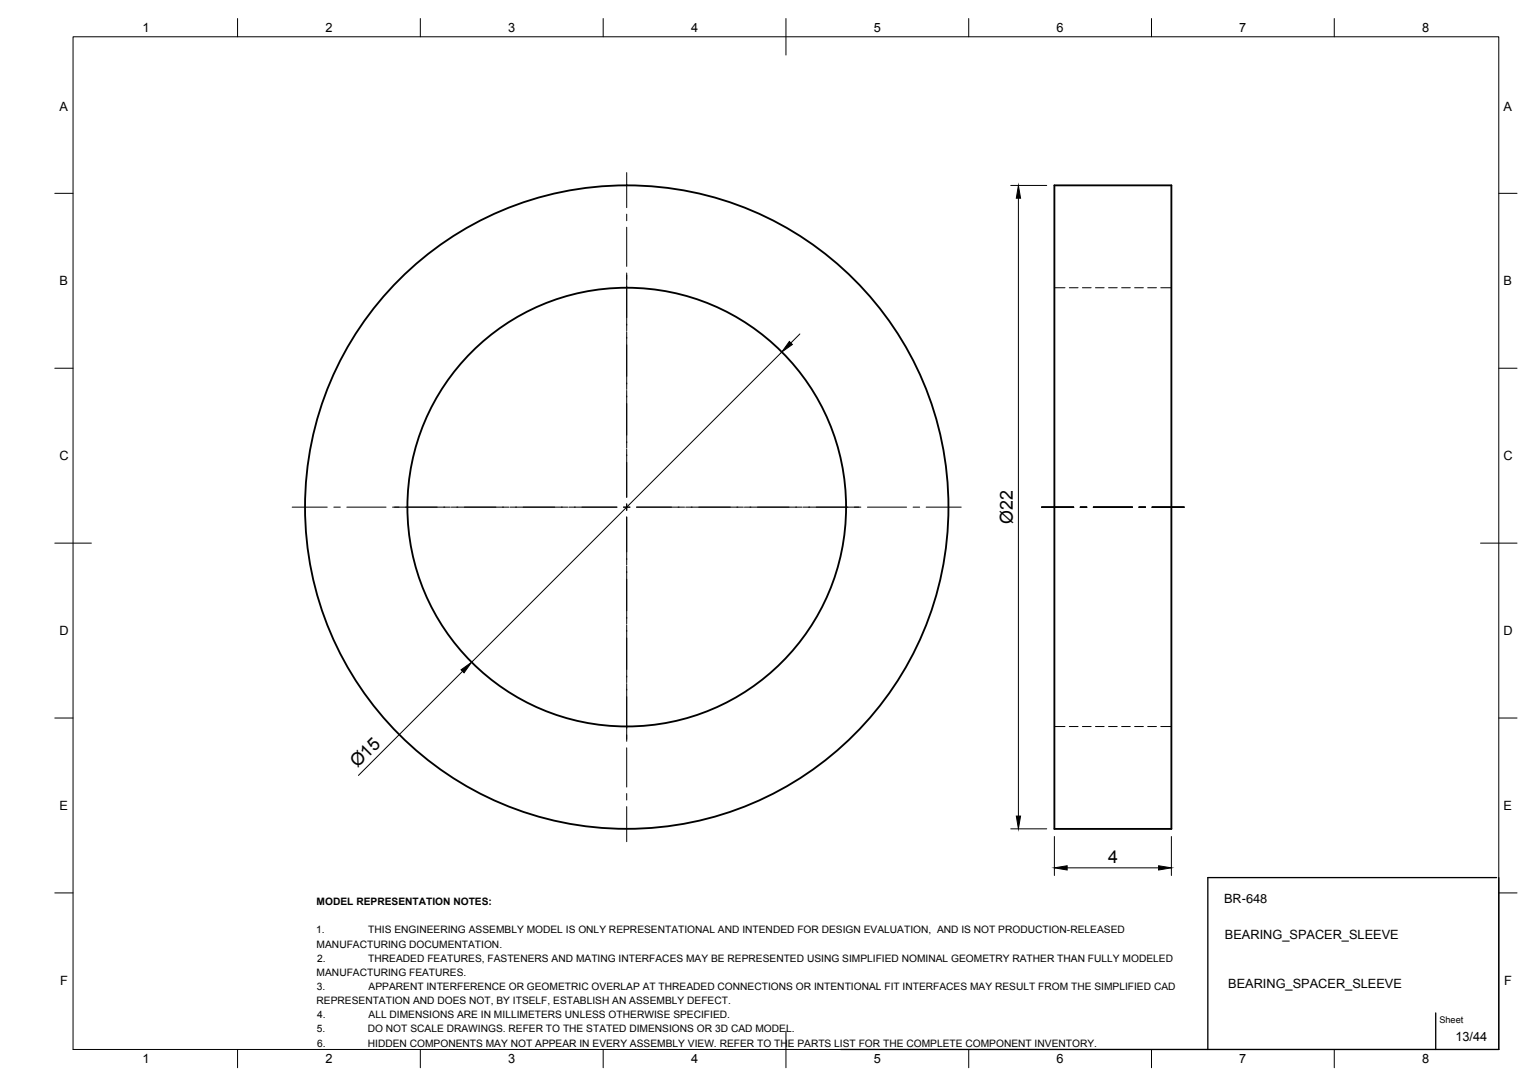
ISO-10303-21;
HEADER;
FILE_DESCRIPTION((''),'2;1');
FILE_NAME('BEARING_SPACER_SLEEVE.step','2026-10-01T22:05:39-07:00',(''),(''),'','','');
FILE_SCHEMA (('AUTOMOTIVE_DESIGN { 1 0 10303 214 3 1 1 }'));
ENDSEC;
DATA;
#10=MECHANICAL_DESIGN_GEOMETRIC_PRESENTATION_REPRESENTATION('',(#613),#24628);
#529=SHAPE_REPRESENTATION_RELATIONSHIP('SRR','None',#24801,#571) ;
#571=ADVANCED_BREP_SHAPE_REPRESENTATION('',(#653),#24591) ;
#613=STYLED_ITEM('',(#25030),#653) ;
#653=MANIFOLD_SOLID_BREP('BEARING_SPACER_SLEEVE',#13124) ;
#847=FACE_BOUND('',#4071,.T.) ;
#848=FACE_BOUND('',#4073,.T.) ;
#1150=LINE('',#20672,#1986) ;
#1151=LINE('',#20678,#1987) ;
#1986=VECTOR('',#16431,0.75) ;
#1987=VECTOR('',#16438,1.1) ;
#2786=CYLINDRICAL_SURFACE('',#14096,0.75) ;
#2787=CYLINDRICAL_SURFACE('',#14099,1.1) ;
#3140=FACE_OUTER_BOUND('',#4068,.T.) ;
#3141=FACE_OUTER_BOUND('',#4069,.T.) ;
#3142=FACE_OUTER_BOUND('',#4070,.T.) ;
#3143=FACE_OUTER_BOUND('',#4072,.T.) ;
#4068=EDGE_LOOP('',(#9285,#9286,#9287,#9288)) ;
#4069=EDGE_LOOP('',(#9289,#9290,#9291,#9292)) ;
#4070=EDGE_LOOP('',(#9293)) ;
#4071=EDGE_LOOP('',(#9294)) ;
#4072=EDGE_LOOP('',(#9295)) ;
#4073=EDGE_LOOP('',(#9296)) ;
#4996=CIRCLE('',#14097,0.75) ;
#4997=CIRCLE('',#14098,0.75) ;
#4998=CIRCLE('',#14100,1.1) ;
#4999=CIRCLE('',#14101,1.1) ;
#5803=VERTEX_POINT('',#20669) ;
#5804=VERTEX_POINT('',#20671) ;
#5805=VERTEX_POINT('',#20675) ;
#5806=VERTEX_POINT('',#20677) ;
#7132=EDGE_CURVE('',#5803,#5803,#4996,.T.) ;
#7133=EDGE_CURVE('',#5803,#5804,#1150,.T.) ;
#7134=EDGE_CURVE('',#5804,#5804,#4997,.T.) ;
#7135=EDGE_CURVE('',#5805,#5805,#4998,.T.) ;
#7136=EDGE_CURVE('',#5805,#5806,#1151,.T.) ;
#7137=EDGE_CURVE('',#5806,#5806,#4999,.T.) ;
#9285=ORIENTED_EDGE('',*,*,#7132,.F.) ;
#9286=ORIENTED_EDGE('',*,*,#7133,.T.) ;
#9287=ORIENTED_EDGE('',*,*,#7134,.F.) ;
#9288=ORIENTED_EDGE('',*,*,#7133,.F.) ;
#9289=ORIENTED_EDGE('',*,*,#7135,.F.) ;
#9290=ORIENTED_EDGE('',*,*,#7136,.T.) ;
#9291=ORIENTED_EDGE('',*,*,#7137,.F.) ;
#9292=ORIENTED_EDGE('',*,*,#7136,.F.) ;
#9293=ORIENTED_EDGE('',*,*,#7137,.T.) ;
#9294=ORIENTED_EDGE('',*,*,#7132,.T.) ;
#9295=ORIENTED_EDGE('',*,*,#7135,.T.) ;
#9296=ORIENTED_EDGE('',*,*,#7134,.T.) ;
#12070=PLANE('',#14102) ;
#12071=PLANE('',#14103) ;
#12535=ADVANCED_FACE('',(#3140),#2786,.F.) ;
#12536=ADVANCED_FACE('',(#3141),#2787,.T.) ;
#12537=ADVANCED_FACE('',(#3142,#847),#12070,.T.) ;
#12538=ADVANCED_FACE('',(#3143,#848),#12071,.T.) ;
#13124=CLOSED_SHELL('',(#12535,#12536,#12537,#12538)) ;
#14095=AXIS2_PLACEMENT_3D('',#20667,#16425,#16426) ;
#14096=AXIS2_PLACEMENT_3D('',#20668,#16427,#16428) ;
#14097=AXIS2_PLACEMENT_3D('',#20670,#16429,#16430) ;
#14098=AXIS2_PLACEMENT_3D('',#20673,#16432,#16433) ;
#14099=AXIS2_PLACEMENT_3D('',#20674,#16434,#16435) ;
#14100=AXIS2_PLACEMENT_3D('',#20676,#16436,#16437) ;
#14101=AXIS2_PLACEMENT_3D('',#20679,#16439,#16440) ;
#14102=AXIS2_PLACEMENT_3D('',#20680,#16441,#16442) ;
#14103=AXIS2_PLACEMENT_3D('',#20681,#16443,#16444) ;
#16425=DIRECTION('axis',(0.,0.,1.)) ;
#16426=DIRECTION('refdir',(1.,0.,0.)) ;
#16427=DIRECTION('center_axis',(0.,1.,0.)) ;
#16428=DIRECTION('ref_axis',(1.,0.,0.)) ;
#16429=DIRECTION('center_axis',(0.,1.,0.)) ;
#16430=DIRECTION('ref_axis',(1.,0.,0.)) ;
#16431=DIRECTION('',(0.,1.,0.)) ;
#16432=DIRECTION('center_axis',(0.,-1.,0.)) ;
#16433=DIRECTION('ref_axis',(1.,0.,0.)) ;
#16434=DIRECTION('center_axis',(0.,1.,0.)) ;
#16435=DIRECTION('ref_axis',(1.,0.,0.)) ;
#16436=DIRECTION('center_axis',(0.,1.,0.)) ;
#16437=DIRECTION('ref_axis',(1.,0.,0.)) ;
#16438=DIRECTION('',(0.,-1.,0.)) ;
#16439=DIRECTION('center_axis',(0.,-1.,0.)) ;
#16440=DIRECTION('ref_axis',(1.,0.,0.)) ;
#16441=DIRECTION('center_axis',(0.,-1.,0.)) ;
#16442=DIRECTION('ref_axis',(-1.,0.,0.)) ;
#16443=DIRECTION('center_axis',(0.,1.,0.)) ;
#16444=DIRECTION('ref_axis',(1.,0.,0.)) ;
#20667=CARTESIAN_POINT('',(0.,0.,0.)) ;
#20668=CARTESIAN_POINT('Origin',(0.,-3.8,0.)) ;
#20669=CARTESIAN_POINT('',(-0.75,-4.,9.18485099360515E-17)) ;
#20670=CARTESIAN_POINT('Origin',(0.,-4.,0.)) ;
#20671=CARTESIAN_POINT('',(-0.75,-3.6,-9.18485099360515E-17)) ;
#20672=CARTESIAN_POINT('',(-0.75,-3.8,9.18485099360515E-17)) ;
#20673=CARTESIAN_POINT('Origin',(0.,-3.6,0.)) ;
#20674=CARTESIAN_POINT('Origin',(0.,-3.8,0.)) ;
#20675=CARTESIAN_POINT('',(-1.1,-3.6,1.34711147906209E-16)) ;
#20676=CARTESIAN_POINT('Origin',(0.,-3.6,0.)) ;
#20677=CARTESIAN_POINT('',(-1.1,-4.,1.34711147906209E-16)) ;
#20678=CARTESIAN_POINT('',(-1.1,-3.8,1.34711147906209E-16)) ;
#20679=CARTESIAN_POINT('Origin',(0.,-4.,0.)) ;
#20680=CARTESIAN_POINT('Origin',(0.,-4.,0.)) ;
#20681=CARTESIAN_POINT('Origin',(0.,-3.6,0.)) ;
#24543=UNCERTAINTY_MEASURE_WITH_UNIT(LENGTH_MEASURE(0.001),#24629,
'DISTANCE_ACCURACY_VALUE',
'Maximum model space distance between geometric entities at asserted c
onnectivities') ;
#24580=UNCERTAINTY_MEASURE_WITH_UNIT(LENGTH_MEASURE(0.001),#24629,
'DISTANCE_ACCURACY_VALUE',
'Maximum model space distance between geometric entities at asserted c
onnectivities') ;
#24591=(
GEOMETRIC_REPRESENTATION_CONTEXT(3)
GLOBAL_UNCERTAINTY_ASSIGNED_CONTEXT((#24543))
GLOBAL_UNIT_ASSIGNED_CONTEXT((#24629,#24631,#24632))
REPRESENTATION_CONTEXT('','3D')
) ;
#24628=(
GEOMETRIC_REPRESENTATION_CONTEXT(3)
GLOBAL_UNCERTAINTY_ASSIGNED_CONTEXT((#24580))
GLOBAL_UNIT_ASSIGNED_CONTEXT((#24629,#24631,#24632))
REPRESENTATION_CONTEXT('','3D')
) ;
#24629=(
LENGTH_UNIT()
NAMED_UNIT(*)
SI_UNIT(.CENTI.,.METRE.)
) ;
#24631=(
NAMED_UNIT(*)
PLANE_ANGLE_UNIT()
SI_UNIT($,.RADIAN.)
) ;
#24632=(
NAMED_UNIT(*)
SI_UNIT($,.STERADIAN.)
SOLID_ANGLE_UNIT()
) ;
#24643=SHAPE_DEFINITION_REPRESENTATION(#24690,#24801) ;
#24690=PRODUCT_DEFINITION_SHAPE('',$,#24849) ;
#24801=SHAPE_REPRESENTATION('',(#14095),#24591) ;
#24838=PRODUCT_DEFINITION_CONTEXT('part definition',#24981,'design') ;
#24849=PRODUCT_DEFINITION('BEARING_SPACER_SLEEVE',
'BEARING_SPACER_SLEEVE',#24896,#24838) ;
#24896=PRODUCT_DEFINITION_FORMATION('',$,#24993) ;
#24981=APPLICATION_CONTEXT(
'Core Data for Automotive Mechanical Design Process') ;
#24982=PRODUCT_CONTEXT('part definition',#24981,'mechanical') ;
#24993=PRODUCT('BEARING_SPACER_SLEEVE','BEARING_SPACER_SLEEVE',$,(#24982)) ;
#25030=PRESENTATION_STYLE_ASSIGNMENT((#25040)) ;
#25040=SURFACE_STYLE_USAGE(.BOTH.,#25050) ;
#25050=SURFACE_SIDE_STYLE('',(#25060)) ;
#25060=SURFACE_STYLE_FILL_AREA(#25070) ;
#25070=FILL_AREA_STYLE('Steel - Satin',(#25080)) ;
#25080=FILL_AREA_STYLE_COLOUR('Steel - Satin',#25090) ;
#25090=COLOUR_RGB('Steel - Satin', 0.66274510, 0.83137255, 0.94901961) ;
ENDSEC;
END-ISO-10303-21;
